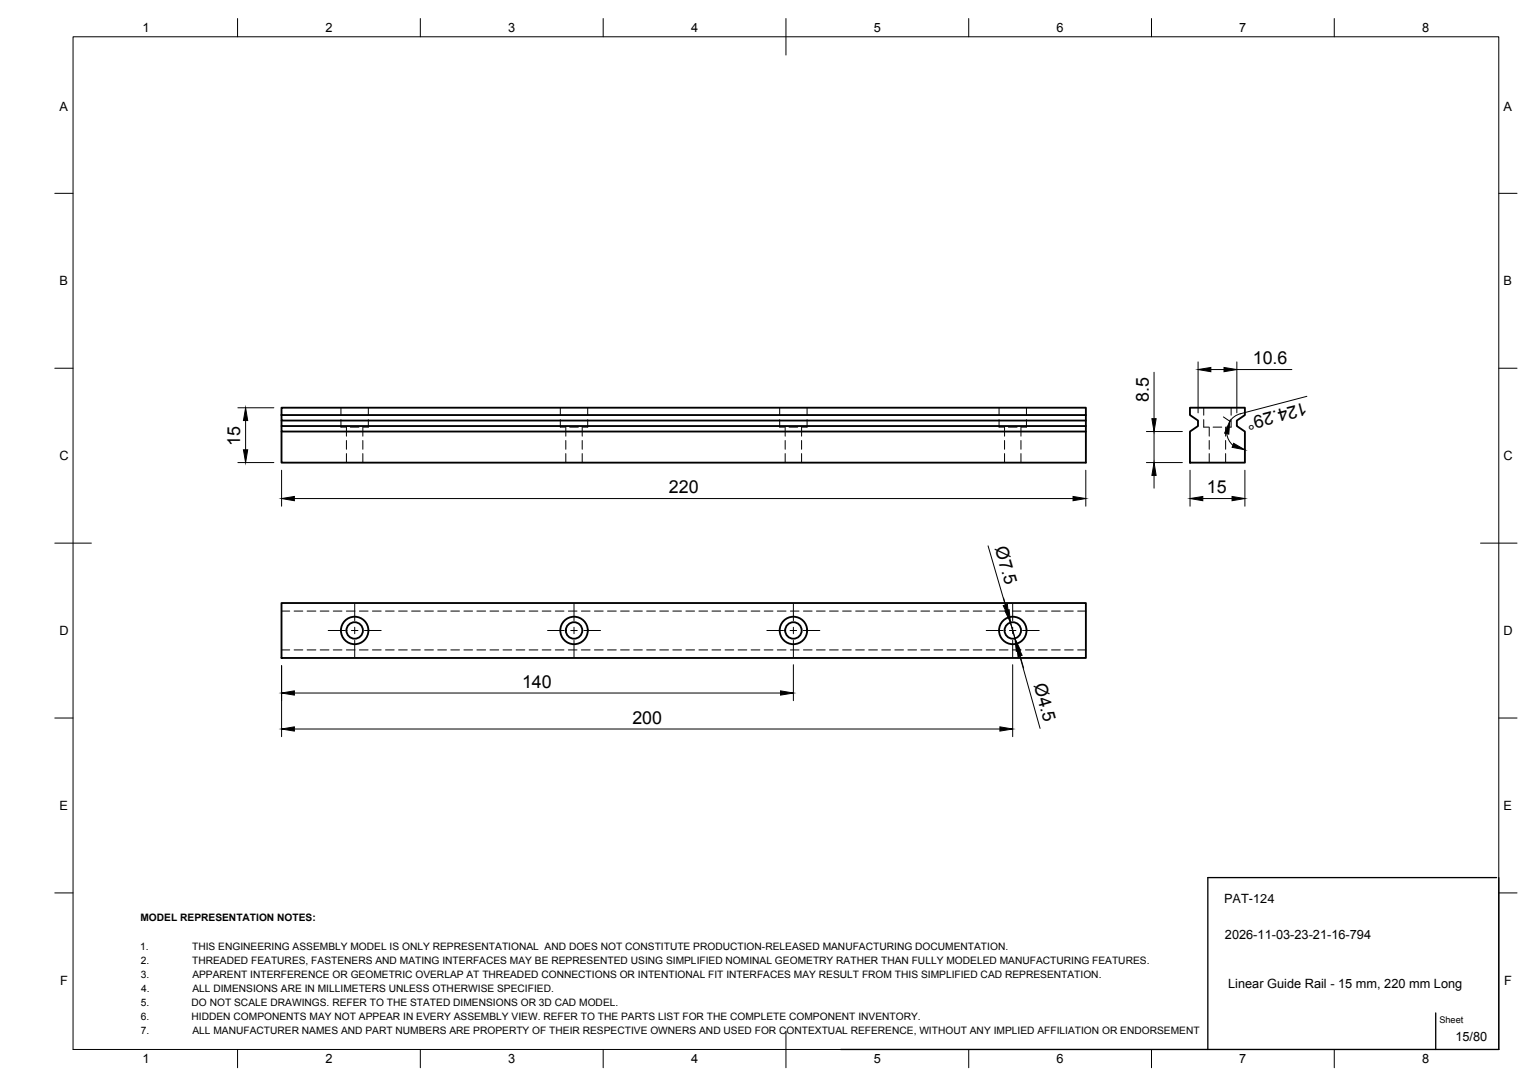
ISO-10303-21;
HEADER;
/* Generated by software containing ST-Developer
 * from STEP Tools, Inc. (www.steptools.com) 
 */

FILE_DESCRIPTION(
/* description */ ('XY cross-slide table'),
/* implementation_level */ '2;1');

FILE_NAME(
/* name */ 'Linear Guide Rail - 15 mm, 220 mm Long.step',
/* time_stamp */ '2026-10-28T03:22:46-07:00',
/* author */ (''),
/* organization */ (''),
/* preprocessor_version */ 'ST-DEVELOPER v20.2',
/* originating_system */ 'Autodesk Translation Framework v15.17.0.0',
/* authorisation */ '');

FILE_SCHEMA (('AUTOMOTIVE_DESIGN { 1 0 10303 214 3 1 1 }'));
ENDSEC;

DATA;
#10=MECHANICAL_DESIGN_GEOMETRIC_PRESENTATION_REPRESENTATION('',(#1680),#62984);
#1514=SHAPE_REPRESENTATION_RELATIONSHIP('SRR','None',#63362,#1597);
#1597=ADVANCED_BREP_SHAPE_REPRESENTATION('',(#1793),#62899);
#1680=STYLED_ITEM('',(#63905),#1793);
#1793=MANIFOLD_SOLID_BREP('Body1',#22974);
#1971=FACE_BOUND('',#4390,.T.);
#1972=FACE_BOUND('',#4393,.T.);
#1973=FACE_BOUND('',#4396,.T.);
#1974=FACE_BOUND('',#4399,.T.);
#1975=FACE_BOUND('',#4409,.T.);
#1976=FACE_BOUND('',#4410,.T.);
#1977=FACE_BOUND('',#4411,.T.);
#1978=FACE_BOUND('',#4412,.T.);
#1979=FACE_BOUND('',#4419,.T.);
#1980=FACE_BOUND('',#4420,.T.);
#1981=FACE_BOUND('',#4421,.T.);
#1982=FACE_BOUND('',#4422,.T.);
#2363=PLANE('',#24246);
#2364=PLANE('',#24251);
#2365=PLANE('',#24256);
#2366=PLANE('',#24261);
#2367=PLANE('',#24271);
#2368=PLANE('',#24272);
#2369=PLANE('',#24273);
#2370=PLANE('',#24274);
#2371=PLANE('',#24275);
#2372=PLANE('',#24276);
#2373=PLANE('',#24277);
#2374=PLANE('',#24278);
#2375=PLANE('',#24279);
#2376=PLANE('',#24280);
#2377=PLANE('',#24281);
#2378=PLANE('',#24282);
#2379=PLANE('',#24283);
#2380=PLANE('',#24284);
#2990=FACE_OUTER_BOUND('',#4388,.T.);
#2991=FACE_OUTER_BOUND('',#4389,.T.);
#2992=FACE_OUTER_BOUND('',#4391,.T.);
#2993=FACE_OUTER_BOUND('',#4392,.T.);
#2994=FACE_OUTER_BOUND('',#4394,.T.);
#2995=FACE_OUTER_BOUND('',#4395,.T.);
#2996=FACE_OUTER_BOUND('',#4397,.T.);
#2997=FACE_OUTER_BOUND('',#4398,.T.);
#2998=FACE_OUTER_BOUND('',#4400,.T.);
#2999=FACE_OUTER_BOUND('',#4401,.T.);
#3000=FACE_OUTER_BOUND('',#4402,.T.);
#3001=FACE_OUTER_BOUND('',#4403,.T.);
#3002=FACE_OUTER_BOUND('',#4404,.T.);
#3003=FACE_OUTER_BOUND('',#4405,.T.);
#3004=FACE_OUTER_BOUND('',#4406,.T.);
#3005=FACE_OUTER_BOUND('',#4407,.T.);
#3006=FACE_OUTER_BOUND('',#4408,.T.);
#3007=FACE_OUTER_BOUND('',#4413,.T.);
#3008=FACE_OUTER_BOUND('',#4414,.T.);
#3009=FACE_OUTER_BOUND('',#4415,.T.);
#3010=FACE_OUTER_BOUND('',#4416,.T.);
#3011=FACE_OUTER_BOUND('',#4417,.T.);
#3012=FACE_OUTER_BOUND('',#4418,.T.);
#3013=FACE_OUTER_BOUND('',#4423,.T.);
#3014=FACE_OUTER_BOUND('',#4424,.T.);
#3015=FACE_OUTER_BOUND('',#4425,.T.);
#4388=EDGE_LOOP('',(#15434,#15435,#15436,#15437));
#4389=EDGE_LOOP('',(#15438));
#4390=EDGE_LOOP('',(#15439));
#4391=EDGE_LOOP('',(#15440,#15441,#15442,#15443));
#4392=EDGE_LOOP('',(#15444));
#4393=EDGE_LOOP('',(#15445));
#4394=EDGE_LOOP('',(#15446,#15447,#15448,#15449));
#4395=EDGE_LOOP('',(#15450));
#4396=EDGE_LOOP('',(#15451));
#4397=EDGE_LOOP('',(#15452,#15453,#15454,#15455));
#4398=EDGE_LOOP('',(#15456));
#4399=EDGE_LOOP('',(#15457));
#4400=EDGE_LOOP('',(#15458,#15459,#15460,#15461));
#4401=EDGE_LOOP('',(#15462,#15463,#15464,#15465));
#4402=EDGE_LOOP('',(#15466,#15467,#15468,#15469));
#4403=EDGE_LOOP('',(#15470,#15471,#15472,#15473));
#4404=EDGE_LOOP('',(#15474,#15475,#15476,#15477));
#4405=EDGE_LOOP('',(#15478,#15479,#15480,#15481));
#4406=EDGE_LOOP('',(#15482,#15483,#15484,#15485));
#4407=EDGE_LOOP('',(#15486,#15487,#15488,#15489));
#4408=EDGE_LOOP('',(#15490,#15491,#15492,#15493));
#4409=EDGE_LOOP('',(#15494));
#4410=EDGE_LOOP('',(#15495));
#4411=EDGE_LOOP('',(#15496));
#4412=EDGE_LOOP('',(#15497));
#4413=EDGE_LOOP('',(#15498,#15499,#15500,#15501));
#4414=EDGE_LOOP('',(#15502,#15503,#15504,#15505));
#4415=EDGE_LOOP('',(#15506,#15507,#15508,#15509));
#4416=EDGE_LOOP('',(#15510,#15511,#15512,#15513));
#4417=EDGE_LOOP('',(#15514,#15515,#15516,#15517));
#4418=EDGE_LOOP('',(#15518,#15519,#15520,#15521));
#4419=EDGE_LOOP('',(#15522));
#4420=EDGE_LOOP('',(#15523));
#4421=EDGE_LOOP('',(#15524));
#4422=EDGE_LOOP('',(#15525));
#4423=EDGE_LOOP('',(#15526,#15527,#15528,#15529));
#4424=EDGE_LOOP('',(#15530,#15531,#15532,#15533,#15534,#15535,#15536,#15537,
#15538,#15539,#15540,#15541));
#4425=EDGE_LOOP('',(#15542,#15543,#15544,#15545,#15546,#15547,#15548,#15549,
#15550,#15551,#15552,#15553));
#6063=LINE('',#33448,#7550);
#6064=LINE('',#33457,#7551);
#6065=LINE('',#33466,#7552);
#6066=LINE('',#33475,#7553);
#6067=LINE('',#33483,#7554);
#6068=LINE('',#33487,#7555);
#6069=LINE('',#33491,#7556);
#6070=LINE('',#33495,#7557);
#6071=LINE('',#33499,#7558);
#6072=LINE('',#33501,#7559);
#6073=LINE('',#33503,#7560);
#6074=LINE('',#33504,#7561);
#6075=LINE('',#33507,#7562);
#6076=LINE('',#33509,#7563);
#6077=LINE('',#33510,#7564);
#6078=LINE('',#33513,#7565);
#6079=LINE('',#33515,#7566);
#6080=LINE('',#33516,#7567);
#6081=LINE('',#33519,#7568);
#6082=LINE('',#33521,#7569);
#6083=LINE('',#33522,#7570);
#6084=LINE('',#33525,#7571);
#6085=LINE('',#33527,#7572);
#6086=LINE('',#33528,#7573);
#6087=LINE('',#33531,#7574);
#6088=LINE('',#33533,#7575);
#6089=LINE('',#33534,#7576);
#6090=LINE('',#33537,#7577);
#6091=LINE('',#33539,#7578);
#6092=LINE('',#33540,#7579);
#6093=LINE('',#33543,#7580);
#6094=LINE('',#33545,#7581);
#6095=LINE('',#33546,#7582);
#6096=LINE('',#33549,#7583);
#6097=LINE('',#33551,#7584);
#6098=LINE('',#33552,#7585);
#6099=LINE('',#33555,#7586);
#6100=LINE('',#33557,#7587);
#6101=LINE('',#33558,#7588);
#6102=LINE('',#33561,#7589);
#6103=LINE('',#33563,#7590);
#6104=LINE('',#33564,#7591);
#6105=LINE('',#33566,#7592);
#6106=LINE('',#33567,#7593);
#7550=VECTOR('',#27108,0.375);
#7551=VECTOR('',#27119,0.375);
#7552=VECTOR('',#27130,0.375);
#7553=VECTOR('',#27141,0.375);
#7554=VECTOR('',#27152,0.225);
#7555=VECTOR('',#27157,0.225);
#7556=VECTOR('',#27162,0.225);
#7557=VECTOR('',#27167,0.225000000000001);
#7558=VECTOR('',#27170,1.);
#7559=VECTOR('',#27171,1.);
#7560=VECTOR('',#27172,1.);
#7561=VECTOR('',#27173,1.);
#7562=VECTOR('',#27176,1.);
#7563=VECTOR('',#27177,1.);
#7564=VECTOR('',#27178,1.);
#7565=VECTOR('',#27181,1.);
#7566=VECTOR('',#27182,1.);
#7567=VECTOR('',#27183,1.);
#7568=VECTOR('',#27186,1.);
#7569=VECTOR('',#27187,1.);
#7570=VECTOR('',#27188,1.);
#7571=VECTOR('',#27191,1.);
#7572=VECTOR('',#27192,1.);
#7573=VECTOR('',#27193,1.);
#7574=VECTOR('',#27196,1.);
#7575=VECTOR('',#27197,1.);
#7576=VECTOR('',#27198,1.);
#7577=VECTOR('',#27201,1.);
#7578=VECTOR('',#27202,1.);
#7579=VECTOR('',#27203,1.);
#7580=VECTOR('',#27206,1.);
#7581=VECTOR('',#27207,1.);
#7582=VECTOR('',#27208,1.);
#7583=VECTOR('',#27211,1.);
#7584=VECTOR('',#27212,1.);
#7585=VECTOR('',#27213,1.);
#7586=VECTOR('',#27216,1.);
#7587=VECTOR('',#27217,1.);
#7588=VECTOR('',#27218,1.);
#7589=VECTOR('',#27221,1.);
#7590=VECTOR('',#27222,1.);
#7591=VECTOR('',#27223,1.);
#7592=VECTOR('',#27226,1.);
#7593=VECTOR('',#27227,1.);
#8988=CIRCLE('',#24244,0.375);
#8989=CIRCLE('',#24245,0.375);
#8990=CIRCLE('',#24247,0.225);
#8991=CIRCLE('',#24249,0.375);
#8992=CIRCLE('',#24250,0.375);
#8993=CIRCLE('',#24252,0.225);
#8994=CIRCLE('',#24254,0.375);
#8995=CIRCLE('',#24255,0.375);
#8996=CIRCLE('',#24257,0.225);
#8997=CIRCLE('',#24259,0.375);
#8998=CIRCLE('',#24260,0.375);
#8999=CIRCLE('',#24262,0.225000000000001);
#9000=CIRCLE('',#24264,0.225);
#9001=CIRCLE('',#24266,0.225);
#9002=CIRCLE('',#24268,0.225);
#9003=CIRCLE('',#24270,0.225000000000001);
#9947=VERTEX_POINT('',#33445);
#9948=VERTEX_POINT('',#33447);
#9949=VERTEX_POINT('',#33451);
#9950=VERTEX_POINT('',#33454);
#9951=VERTEX_POINT('',#33456);
#9952=VERTEX_POINT('',#33460);
#9953=VERTEX_POINT('',#33463);
#9954=VERTEX_POINT('',#33465);
#9955=VERTEX_POINT('',#33469);
#9956=VERTEX_POINT('',#33472);
#9957=VERTEX_POINT('',#33474);
#9958=VERTEX_POINT('',#33478);
#9959=VERTEX_POINT('',#33481);
#9960=VERTEX_POINT('',#33485);
#9961=VERTEX_POINT('',#33489);
#9962=VERTEX_POINT('',#33493);
#9963=VERTEX_POINT('',#33497);
#9964=VERTEX_POINT('',#33498);
#9965=VERTEX_POINT('',#33500);
#9966=VERTEX_POINT('',#33502);
#9967=VERTEX_POINT('',#33506);
#9968=VERTEX_POINT('',#33508);
#9969=VERTEX_POINT('',#33512);
#9970=VERTEX_POINT('',#33514);
#9971=VERTEX_POINT('',#33518);
#9972=VERTEX_POINT('',#33520);
#9973=VERTEX_POINT('',#33524);
#9974=VERTEX_POINT('',#33526);
#9975=VERTEX_POINT('',#33530);
#9976=VERTEX_POINT('',#33532);
#9977=VERTEX_POINT('',#33536);
#9978=VERTEX_POINT('',#33538);
#9979=VERTEX_POINT('',#33542);
#9980=VERTEX_POINT('',#33544);
#9981=VERTEX_POINT('',#33548);
#9982=VERTEX_POINT('',#33550);
#9983=VERTEX_POINT('',#33554);
#9984=VERTEX_POINT('',#33556);
#9985=VERTEX_POINT('',#33560);
#9986=VERTEX_POINT('',#33562);
#12101=EDGE_CURVE('',#9947,#9947,#8988,.T.);
#12102=EDGE_CURVE('',#9947,#9948,#6063,.T.);
#12103=EDGE_CURVE('',#9948,#9948,#8989,.T.);
#12104=EDGE_CURVE('',#9949,#9949,#8990,.T.);
#12105=EDGE_CURVE('',#9950,#9950,#8991,.T.);
#12106=EDGE_CURVE('',#9950,#9951,#6064,.T.);
#12107=EDGE_CURVE('',#9951,#9951,#8992,.T.);
#12108=EDGE_CURVE('',#9952,#9952,#8993,.T.);
#12109=EDGE_CURVE('',#9953,#9953,#8994,.T.);
#12110=EDGE_CURVE('',#9953,#9954,#6065,.T.);
#12111=EDGE_CURVE('',#9954,#9954,#8995,.T.);
#12112=EDGE_CURVE('',#9955,#9955,#8996,.T.);
#12113=EDGE_CURVE('',#9956,#9956,#8997,.T.);
#12114=EDGE_CURVE('',#9956,#9957,#6066,.T.);
#12115=EDGE_CURVE('',#9957,#9957,#8998,.T.);
#12116=EDGE_CURVE('',#9958,#9958,#8999,.T.);
#12117=EDGE_CURVE('',#9959,#9959,#9000,.T.);
#12118=EDGE_CURVE('',#9959,#9949,#6067,.T.);
#12119=EDGE_CURVE('',#9960,#9960,#9001,.T.);
#12120=EDGE_CURVE('',#9960,#9952,#6068,.T.);
#12121=EDGE_CURVE('',#9961,#9961,#9002,.T.);
#12122=EDGE_CURVE('',#9961,#9955,#6069,.T.);
#12123=EDGE_CURVE('',#9962,#9962,#9003,.T.);
#12124=EDGE_CURVE('',#9962,#9958,#6070,.T.);
#12125=EDGE_CURVE('',#9963,#9964,#6071,.T.);
#12126=EDGE_CURVE('',#9964,#9965,#6072,.T.);
#12127=EDGE_CURVE('',#9966,#9965,#6073,.T.);
#12128=EDGE_CURVE('',#9963,#9966,#6074,.T.);
#12129=EDGE_CURVE('',#9967,#9963,#6075,.T.);
#12130=EDGE_CURVE('',#9968,#9966,#6076,.T.);
#12131=EDGE_CURVE('',#9967,#9968,#6077,.T.);
#12132=EDGE_CURVE('',#9969,#9967,#6078,.T.);
#12133=EDGE_CURVE('',#9970,#9968,#6079,.T.);
#12134=EDGE_CURVE('',#9969,#9970,#6080,.T.);
#12135=EDGE_CURVE('',#9971,#9969,#6081,.T.);
#12136=EDGE_CURVE('',#9972,#9970,#6082,.T.);
#12137=EDGE_CURVE('',#9971,#9972,#6083,.T.);
#12138=EDGE_CURVE('',#9973,#9971,#6084,.T.);
#12139=EDGE_CURVE('',#9974,#9972,#6085,.T.);
#12140=EDGE_CURVE('',#9973,#9974,#6086,.T.);
#12141=EDGE_CURVE('',#9975,#9973,#6087,.T.);
#12142=EDGE_CURVE('',#9976,#9974,#6088,.T.);
#12143=EDGE_CURVE('',#9975,#9976,#6089,.T.);
#12144=EDGE_CURVE('',#9977,#9975,#6090,.T.);
#12145=EDGE_CURVE('',#9978,#9976,#6091,.T.);
#12146=EDGE_CURVE('',#9977,#9978,#6092,.T.);
#12147=EDGE_CURVE('',#9979,#9977,#6093,.T.);
#12148=EDGE_CURVE('',#9980,#9978,#6094,.T.);
#12149=EDGE_CURVE('',#9979,#9980,#6095,.T.);
#12150=EDGE_CURVE('',#9981,#9979,#6096,.T.);
#12151=EDGE_CURVE('',#9982,#9980,#6097,.T.);
#12152=EDGE_CURVE('',#9981,#9982,#6098,.T.);
#12153=EDGE_CURVE('',#9983,#9981,#6099,.T.);
#12154=EDGE_CURVE('',#9984,#9982,#6100,.T.);
#12155=EDGE_CURVE('',#9983,#9984,#6101,.T.);
#12156=EDGE_CURVE('',#9985,#9983,#6102,.T.);
#12157=EDGE_CURVE('',#9986,#9984,#6103,.T.);
#12158=EDGE_CURVE('',#9985,#9986,#6104,.T.);
#12159=EDGE_CURVE('',#9964,#9985,#6105,.T.);
#12160=EDGE_CURVE('',#9965,#9986,#6106,.T.);
#15434=ORIENTED_EDGE('',*,*,#12101,.F.);
#15435=ORIENTED_EDGE('',*,*,#12102,.T.);
#15436=ORIENTED_EDGE('',*,*,#12103,.F.);
#15437=ORIENTED_EDGE('',*,*,#12102,.F.);
#15438=ORIENTED_EDGE('',*,*,#12101,.T.);
#15439=ORIENTED_EDGE('',*,*,#12104,.F.);
#15440=ORIENTED_EDGE('',*,*,#12105,.F.);
#15441=ORIENTED_EDGE('',*,*,#12106,.T.);
#15442=ORIENTED_EDGE('',*,*,#12107,.F.);
#15443=ORIENTED_EDGE('',*,*,#12106,.F.);
#15444=ORIENTED_EDGE('',*,*,#12105,.T.);
#15445=ORIENTED_EDGE('',*,*,#12108,.F.);
#15446=ORIENTED_EDGE('',*,*,#12109,.F.);
#15447=ORIENTED_EDGE('',*,*,#12110,.T.);
#15448=ORIENTED_EDGE('',*,*,#12111,.F.);
#15449=ORIENTED_EDGE('',*,*,#12110,.F.);
#15450=ORIENTED_EDGE('',*,*,#12109,.T.);
#15451=ORIENTED_EDGE('',*,*,#12112,.F.);
#15452=ORIENTED_EDGE('',*,*,#12113,.F.);
#15453=ORIENTED_EDGE('',*,*,#12114,.T.);
#15454=ORIENTED_EDGE('',*,*,#12115,.F.);
#15455=ORIENTED_EDGE('',*,*,#12114,.F.);
#15456=ORIENTED_EDGE('',*,*,#12113,.T.);
#15457=ORIENTED_EDGE('',*,*,#12116,.F.);
#15458=ORIENTED_EDGE('',*,*,#12117,.F.);
#15459=ORIENTED_EDGE('',*,*,#12118,.T.);
#15460=ORIENTED_EDGE('',*,*,#12104,.T.);
#15461=ORIENTED_EDGE('',*,*,#12118,.F.);
#15462=ORIENTED_EDGE('',*,*,#12119,.F.);
#15463=ORIENTED_EDGE('',*,*,#12120,.T.);
#15464=ORIENTED_EDGE('',*,*,#12108,.T.);
#15465=ORIENTED_EDGE('',*,*,#12120,.F.);
#15466=ORIENTED_EDGE('',*,*,#12121,.F.);
#15467=ORIENTED_EDGE('',*,*,#12122,.T.);
#15468=ORIENTED_EDGE('',*,*,#12112,.T.);
#15469=ORIENTED_EDGE('',*,*,#12122,.F.);
#15470=ORIENTED_EDGE('',*,*,#12123,.F.);
#15471=ORIENTED_EDGE('',*,*,#12124,.T.);
#15472=ORIENTED_EDGE('',*,*,#12116,.T.);
#15473=ORIENTED_EDGE('',*,*,#12124,.F.);
#15474=ORIENTED_EDGE('',*,*,#12125,.T.);
#15475=ORIENTED_EDGE('',*,*,#12126,.T.);
#15476=ORIENTED_EDGE('',*,*,#12127,.F.);
#15477=ORIENTED_EDGE('',*,*,#12128,.F.);
#15478=ORIENTED_EDGE('',*,*,#12129,.T.);
#15479=ORIENTED_EDGE('',*,*,#12128,.T.);
#15480=ORIENTED_EDGE('',*,*,#12130,.F.);
#15481=ORIENTED_EDGE('',*,*,#12131,.F.);
#15482=ORIENTED_EDGE('',*,*,#12132,.T.);
#15483=ORIENTED_EDGE('',*,*,#12131,.T.);
#15484=ORIENTED_EDGE('',*,*,#12133,.F.);
#15485=ORIENTED_EDGE('',*,*,#12134,.F.);
#15486=ORIENTED_EDGE('',*,*,#12135,.T.);
#15487=ORIENTED_EDGE('',*,*,#12134,.T.);
#15488=ORIENTED_EDGE('',*,*,#12136,.F.);
#15489=ORIENTED_EDGE('',*,*,#12137,.F.);
#15490=ORIENTED_EDGE('',*,*,#12138,.T.);
#15491=ORIENTED_EDGE('',*,*,#12137,.T.);
#15492=ORIENTED_EDGE('',*,*,#12139,.F.);
#15493=ORIENTED_EDGE('',*,*,#12140,.F.);
#15494=ORIENTED_EDGE('',*,*,#12115,.T.);
#15495=ORIENTED_EDGE('',*,*,#12111,.T.);
#15496=ORIENTED_EDGE('',*,*,#12107,.T.);
#15497=ORIENTED_EDGE('',*,*,#12103,.T.);
#15498=ORIENTED_EDGE('',*,*,#12141,.T.);
#15499=ORIENTED_EDGE('',*,*,#12140,.T.);
#15500=ORIENTED_EDGE('',*,*,#12142,.F.);
#15501=ORIENTED_EDGE('',*,*,#12143,.F.);
#15502=ORIENTED_EDGE('',*,*,#12144,.T.);
#15503=ORIENTED_EDGE('',*,*,#12143,.T.);
#15504=ORIENTED_EDGE('',*,*,#12145,.F.);
#15505=ORIENTED_EDGE('',*,*,#12146,.F.);
#15506=ORIENTED_EDGE('',*,*,#12147,.T.);
#15507=ORIENTED_EDGE('',*,*,#12146,.T.);
#15508=ORIENTED_EDGE('',*,*,#12148,.F.);
#15509=ORIENTED_EDGE('',*,*,#12149,.F.);
#15510=ORIENTED_EDGE('',*,*,#12150,.T.);
#15511=ORIENTED_EDGE('',*,*,#12149,.T.);
#15512=ORIENTED_EDGE('',*,*,#12151,.F.);
#15513=ORIENTED_EDGE('',*,*,#12152,.F.);
#15514=ORIENTED_EDGE('',*,*,#12153,.T.);
#15515=ORIENTED_EDGE('',*,*,#12152,.T.);
#15516=ORIENTED_EDGE('',*,*,#12154,.F.);
#15517=ORIENTED_EDGE('',*,*,#12155,.F.);
#15518=ORIENTED_EDGE('',*,*,#12156,.T.);
#15519=ORIENTED_EDGE('',*,*,#12155,.T.);
#15520=ORIENTED_EDGE('',*,*,#12157,.F.);
#15521=ORIENTED_EDGE('',*,*,#12158,.F.);
#15522=ORIENTED_EDGE('',*,*,#12117,.T.);
#15523=ORIENTED_EDGE('',*,*,#12119,.T.);
#15524=ORIENTED_EDGE('',*,*,#12121,.T.);
#15525=ORIENTED_EDGE('',*,*,#12123,.T.);
#15526=ORIENTED_EDGE('',*,*,#12159,.T.);
#15527=ORIENTED_EDGE('',*,*,#12158,.T.);
#15528=ORIENTED_EDGE('',*,*,#12160,.F.);
#15529=ORIENTED_EDGE('',*,*,#12126,.F.);
#15530=ORIENTED_EDGE('',*,*,#12160,.T.);
#15531=ORIENTED_EDGE('',*,*,#12157,.T.);
#15532=ORIENTED_EDGE('',*,*,#12154,.T.);
#15533=ORIENTED_EDGE('',*,*,#12151,.T.);
#15534=ORIENTED_EDGE('',*,*,#12148,.T.);
#15535=ORIENTED_EDGE('',*,*,#12145,.T.);
#15536=ORIENTED_EDGE('',*,*,#12142,.T.);
#15537=ORIENTED_EDGE('',*,*,#12139,.T.);
#15538=ORIENTED_EDGE('',*,*,#12136,.T.);
#15539=ORIENTED_EDGE('',*,*,#12133,.T.);
#15540=ORIENTED_EDGE('',*,*,#12130,.T.);
#15541=ORIENTED_EDGE('',*,*,#12127,.T.);
#15542=ORIENTED_EDGE('',*,*,#12159,.F.);
#15543=ORIENTED_EDGE('',*,*,#12125,.F.);
#15544=ORIENTED_EDGE('',*,*,#12129,.F.);
#15545=ORIENTED_EDGE('',*,*,#12132,.F.);
#15546=ORIENTED_EDGE('',*,*,#12135,.F.);
#15547=ORIENTED_EDGE('',*,*,#12138,.F.);
#15548=ORIENTED_EDGE('',*,*,#12141,.F.);
#15549=ORIENTED_EDGE('',*,*,#12144,.F.);
#15550=ORIENTED_EDGE('',*,*,#12147,.F.);
#15551=ORIENTED_EDGE('',*,*,#12150,.F.);
#15552=ORIENTED_EDGE('',*,*,#12153,.F.);
#15553=ORIENTED_EDGE('',*,*,#12156,.F.);
#21094=CYLINDRICAL_SURFACE('',#24243,0.375);
#21095=CYLINDRICAL_SURFACE('',#24248,0.375);
#21096=CYLINDRICAL_SURFACE('',#24253,0.375);
#21097=CYLINDRICAL_SURFACE('',#24258,0.375);
#21098=CYLINDRICAL_SURFACE('',#24263,0.225);
#21099=CYLINDRICAL_SURFACE('',#24265,0.225);
#21100=CYLINDRICAL_SURFACE('',#24267,0.225);
#21101=CYLINDRICAL_SURFACE('',#24269,0.225000000000001);
#21771=ADVANCED_FACE('',(#2990),#21094,.F.);
#21772=ADVANCED_FACE('',(#2991,#1971),#2363,.T.);
#21773=ADVANCED_FACE('',(#2992),#21095,.F.);
#21774=ADVANCED_FACE('',(#2993,#1972),#2364,.T.);
#21775=ADVANCED_FACE('',(#2994),#21096,.F.);
#21776=ADVANCED_FACE('',(#2995,#1973),#2365,.T.);
#21777=ADVANCED_FACE('',(#2996),#21097,.F.);
#21778=ADVANCED_FACE('',(#2997,#1974),#2366,.T.);
#21779=ADVANCED_FACE('',(#2998),#21098,.F.);
#21780=ADVANCED_FACE('',(#2999),#21099,.F.);
#21781=ADVANCED_FACE('',(#3000),#21100,.F.);
#21782=ADVANCED_FACE('',(#3001),#21101,.F.);
#21783=ADVANCED_FACE('',(#3002),#2367,.T.);
#21784=ADVANCED_FACE('',(#3003),#2368,.T.);
#21785=ADVANCED_FACE('',(#3004),#2369,.T.);
#21786=ADVANCED_FACE('',(#3005),#2370,.T.);
#21787=ADVANCED_FACE('',(#3006,#1975,#1976,#1977,#1978),#2371,.T.);
#21788=ADVANCED_FACE('',(#3007),#2372,.T.);
#21789=ADVANCED_FACE('',(#3008),#2373,.T.);
#21790=ADVANCED_FACE('',(#3009),#2374,.T.);
#21791=ADVANCED_FACE('',(#3010),#2375,.T.);
#21792=ADVANCED_FACE('',(#3011),#2376,.T.);
#21793=ADVANCED_FACE('',(#3012,#1979,#1980,#1981,#1982),#2377,.T.);
#21794=ADVANCED_FACE('',(#3013),#2378,.T.);
#21795=ADVANCED_FACE('',(#3014),#2379,.T.);
#21796=ADVANCED_FACE('',(#3015),#2380,.F.);
#22974=CLOSED_SHELL('',(#21771,#21772,#21773,#21774,#21775,#21776,#21777,
#21778,#21779,#21780,#21781,#21782,#21783,#21784,#21785,#21786,#21787,#21788,
#21789,#21790,#21791,#21792,#21793,#21794,#21795,#21796));
#24242=AXIS2_PLACEMENT_3D('',#33443,#27102,#27103);
#24243=AXIS2_PLACEMENT_3D('',#33444,#27104,#27105);
#24244=AXIS2_PLACEMENT_3D('',#33446,#27106,#27107);
#24245=AXIS2_PLACEMENT_3D('',#33449,#27109,#27110);
#24246=AXIS2_PLACEMENT_3D('',#33450,#27111,#27112);
#24247=AXIS2_PLACEMENT_3D('',#33452,#27113,#27114);
#24248=AXIS2_PLACEMENT_3D('',#33453,#27115,#27116);
#24249=AXIS2_PLACEMENT_3D('',#33455,#27117,#27118);
#24250=AXIS2_PLACEMENT_3D('',#33458,#27120,#27121);
#24251=AXIS2_PLACEMENT_3D('',#33459,#27122,#27123);
#24252=AXIS2_PLACEMENT_3D('',#33461,#27124,#27125);
#24253=AXIS2_PLACEMENT_3D('',#33462,#27126,#27127);
#24254=AXIS2_PLACEMENT_3D('',#33464,#27128,#27129);
#24255=AXIS2_PLACEMENT_3D('',#33467,#27131,#27132);
#24256=AXIS2_PLACEMENT_3D('',#33468,#27133,#27134);
#24257=AXIS2_PLACEMENT_3D('',#33470,#27135,#27136);
#24258=AXIS2_PLACEMENT_3D('',#33471,#27137,#27138);
#24259=AXIS2_PLACEMENT_3D('',#33473,#27139,#27140);
#24260=AXIS2_PLACEMENT_3D('',#33476,#27142,#27143);
#24261=AXIS2_PLACEMENT_3D('',#33477,#27144,#27145);
#24262=AXIS2_PLACEMENT_3D('',#33479,#27146,#27147);
#24263=AXIS2_PLACEMENT_3D('',#33480,#27148,#27149);
#24264=AXIS2_PLACEMENT_3D('',#33482,#27150,#27151);
#24265=AXIS2_PLACEMENT_3D('',#33484,#27153,#27154);
#24266=AXIS2_PLACEMENT_3D('',#33486,#27155,#27156);
#24267=AXIS2_PLACEMENT_3D('',#33488,#27158,#27159);
#24268=AXIS2_PLACEMENT_3D('',#33490,#27160,#27161);
#24269=AXIS2_PLACEMENT_3D('',#33492,#27163,#27164);
#24270=AXIS2_PLACEMENT_3D('',#33494,#27165,#27166);
#24271=AXIS2_PLACEMENT_3D('',#33496,#27168,#27169);
#24272=AXIS2_PLACEMENT_3D('',#33505,#27174,#27175);
#24273=AXIS2_PLACEMENT_3D('',#33511,#27179,#27180);
#24274=AXIS2_PLACEMENT_3D('',#33517,#27184,#27185);
#24275=AXIS2_PLACEMENT_3D('',#33523,#27189,#27190);
#24276=AXIS2_PLACEMENT_3D('',#33529,#27194,#27195);
#24277=AXIS2_PLACEMENT_3D('',#33535,#27199,#27200);
#24278=AXIS2_PLACEMENT_3D('',#33541,#27204,#27205);
#24279=AXIS2_PLACEMENT_3D('',#33547,#27209,#27210);
#24280=AXIS2_PLACEMENT_3D('',#33553,#27214,#27215);
#24281=AXIS2_PLACEMENT_3D('',#33559,#27219,#27220);
#24282=AXIS2_PLACEMENT_3D('',#33565,#27224,#27225);
#24283=AXIS2_PLACEMENT_3D('',#33568,#27228,#27229);
#24284=AXIS2_PLACEMENT_3D('',#33569,#27230,#27231);
#27102=DIRECTION('axis',(0.,0.,1.));
#27103=DIRECTION('refdir',(1.,0.,0.));
#27104=DIRECTION('center_axis',(0.,0.,1.));
#27105=DIRECTION('ref_axis',(1.,0.,0.));
#27106=DIRECTION('center_axis',(0.,0.,1.));
#27107=DIRECTION('ref_axis',(1.,0.,0.));
#27108=DIRECTION('',(0.,0.,1.));
#27109=DIRECTION('center_axis',(0.,0.,-1.));
#27110=DIRECTION('ref_axis',(1.,0.,0.));
#27111=DIRECTION('center_axis',(0.,0.,1.));
#27112=DIRECTION('ref_axis',(1.,0.,0.));
#27113=DIRECTION('center_axis',(0.,0.,1.));
#27114=DIRECTION('ref_axis',(1.,0.,0.));
#27115=DIRECTION('center_axis',(0.,0.,1.));
#27116=DIRECTION('ref_axis',(1.,0.,0.));
#27117=DIRECTION('center_axis',(0.,0.,1.));
#27118=DIRECTION('ref_axis',(1.,0.,0.));
#27119=DIRECTION('',(0.,0.,1.));
#27120=DIRECTION('center_axis',(0.,0.,-1.));
#27121=DIRECTION('ref_axis',(1.,0.,0.));
#27122=DIRECTION('center_axis',(0.,0.,1.));
#27123=DIRECTION('ref_axis',(1.,0.,0.));
#27124=DIRECTION('center_axis',(0.,0.,1.));
#27125=DIRECTION('ref_axis',(1.,0.,0.));
#27126=DIRECTION('center_axis',(0.,0.,1.));
#27127=DIRECTION('ref_axis',(1.,0.,0.));
#27128=DIRECTION('center_axis',(0.,0.,1.));
#27129=DIRECTION('ref_axis',(1.,0.,0.));
#27130=DIRECTION('',(0.,0.,1.));
#27131=DIRECTION('center_axis',(0.,0.,-1.));
#27132=DIRECTION('ref_axis',(1.,0.,0.));
#27133=DIRECTION('center_axis',(0.,0.,1.));
#27134=DIRECTION('ref_axis',(1.,0.,0.));
#27135=DIRECTION('center_axis',(0.,0.,1.));
#27136=DIRECTION('ref_axis',(1.,0.,0.));
#27137=DIRECTION('center_axis',(0.,0.,1.));
#27138=DIRECTION('ref_axis',(1.,0.,0.));
#27139=DIRECTION('center_axis',(0.,0.,1.));
#27140=DIRECTION('ref_axis',(1.,0.,0.));
#27141=DIRECTION('',(0.,0.,1.));
#27142=DIRECTION('center_axis',(0.,0.,-1.));
#27143=DIRECTION('ref_axis',(1.,0.,0.));
#27144=DIRECTION('center_axis',(0.,0.,1.));
#27145=DIRECTION('ref_axis',(1.,0.,0.));
#27146=DIRECTION('center_axis',(0.,0.,1.));
#27147=DIRECTION('ref_axis',(1.,0.,0.));
#27148=DIRECTION('center_axis',(0.,0.,1.));
#27149=DIRECTION('ref_axis',(1.,0.,0.));
#27150=DIRECTION('center_axis',(0.,0.,1.));
#27151=DIRECTION('ref_axis',(1.,0.,0.));
#27152=DIRECTION('',(0.,0.,1.));
#27153=DIRECTION('center_axis',(0.,0.,1.));
#27154=DIRECTION('ref_axis',(1.,0.,0.));
#27155=DIRECTION('center_axis',(0.,0.,1.));
#27156=DIRECTION('ref_axis',(1.,0.,0.));
#27157=DIRECTION('',(0.,0.,1.));
#27158=DIRECTION('center_axis',(0.,0.,1.));
#27159=DIRECTION('ref_axis',(1.,0.,0.));
#27160=DIRECTION('center_axis',(0.,0.,1.));
#27161=DIRECTION('ref_axis',(1.,0.,0.));
#27162=DIRECTION('',(0.,0.,1.));
#27163=DIRECTION('center_axis',(0.,0.,1.));
#27164=DIRECTION('ref_axis',(1.,0.,0.));
#27165=DIRECTION('center_axis',(0.,0.,1.));
#27166=DIRECTION('ref_axis',(1.,0.,0.));
#27167=DIRECTION('',(0.,0.,1.));
#27168=DIRECTION('center_axis',(0.,-0.56333682464151,0.826227342807548));
#27169=DIRECTION('ref_axis',(0.,-0.826227342807548,-0.56333682464151));
#27170=DIRECTION('',(0.,-0.826227342807548,-0.56333682464151));
#27171=DIRECTION('',(1.,0.,0.));
#27172=DIRECTION('',(0.,-0.826227342807548,-0.56333682464151));
#27173=DIRECTION('',(1.,0.,0.));
#27174=DIRECTION('center_axis',(0.,-1.,0.));
#27175=DIRECTION('ref_axis',(0.,0.,-1.));
#27176=DIRECTION('',(0.,0.,-1.));
#27177=DIRECTION('',(0.,0.,-1.));
#27178=DIRECTION('',(1.,0.,0.));
#27179=DIRECTION('center_axis',(0.,-0.56333682464151,-0.826227342807548));
#27180=DIRECTION('ref_axis',(0.,0.826227342807548,-0.56333682464151));
#27181=DIRECTION('',(0.,0.826227342807548,-0.56333682464151));
#27182=DIRECTION('',(0.,0.826227342807548,-0.56333682464151));
#27183=DIRECTION('',(1.,0.,0.));
#27184=DIRECTION('center_axis',(0.,-1.,0.));
#27185=DIRECTION('ref_axis',(0.,0.,-1.));
#27186=DIRECTION('',(0.,0.,-1.));
#27187=DIRECTION('',(0.,0.,-1.));
#27188=DIRECTION('',(1.,0.,0.));
#27189=DIRECTION('center_axis',(0.,0.,1.));
#27190=DIRECTION('ref_axis',(0.,-1.,0.));
#27191=DIRECTION('',(0.,-1.,0.));
#27192=DIRECTION('',(0.,-1.,0.));
#27193=DIRECTION('',(1.,0.,0.));
#27194=DIRECTION('center_axis',(0.,1.,0.));
#27195=DIRECTION('ref_axis',(0.,0.,1.));
#27196=DIRECTION('',(0.,0.,1.));
#27197=DIRECTION('',(0.,0.,1.));
#27198=DIRECTION('',(1.,0.,0.));
#27199=DIRECTION('center_axis',(0.,0.56333682464151,-0.826227342807548));
#27200=DIRECTION('ref_axis',(0.,0.826227342807548,0.56333682464151));
#27201=DIRECTION('',(0.,0.826227342807548,0.56333682464151));
#27202=DIRECTION('',(0.,0.826227342807548,0.56333682464151));
#27203=DIRECTION('',(1.,0.,0.));
#27204=DIRECTION('center_axis',(0.,1.,0.));
#27205=DIRECTION('ref_axis',(0.,0.,1.));
#27206=DIRECTION('',(0.,0.,1.));
#27207=DIRECTION('',(0.,0.,1.));
#27208=DIRECTION('',(1.,0.,0.));
#27209=DIRECTION('center_axis',(0.,0.56333682464151,0.826227342807548));
#27210=DIRECTION('ref_axis',(0.,-0.826227342807548,0.56333682464151));
#27211=DIRECTION('',(0.,-0.826227342807548,0.56333682464151));
#27212=DIRECTION('',(0.,-0.826227342807548,0.56333682464151));
#27213=DIRECTION('',(1.,0.,0.));
#27214=DIRECTION('center_axis',(0.,1.,0.));
#27215=DIRECTION('ref_axis',(0.,0.,1.));
#27216=DIRECTION('',(0.,0.,1.));
#27217=DIRECTION('',(0.,0.,1.));
#27218=DIRECTION('',(1.,0.,0.));
#27219=DIRECTION('center_axis',(0.,0.,-1.));
#27220=DIRECTION('ref_axis',(0.,1.,0.));
#27221=DIRECTION('',(0.,1.,0.));
#27222=DIRECTION('',(0.,1.,0.));
#27223=DIRECTION('',(1.,0.,0.));
#27224=DIRECTION('center_axis',(0.,-1.,0.));
#27225=DIRECTION('ref_axis',(0.,0.,-1.));
#27226=DIRECTION('',(0.,0.,-1.));
#27227=DIRECTION('',(0.,0.,-1.));
#27228=DIRECTION('center_axis',(1.,0.,0.));
#27229=DIRECTION('ref_axis',(0.,0.,-1.));
#27230=DIRECTION('center_axis',(1.,0.,0.));
#27231=DIRECTION('ref_axis',(0.,0.,-1.));
#33443=CARTESIAN_POINT('',(0.,0.,0.));
#33444=CARTESIAN_POINT('Origin',(14.,0.,0.97));
#33445=CARTESIAN_POINT('',(13.625,-4.59242549680257E-17,0.97));
#33446=CARTESIAN_POINT('Origin',(14.,0.,0.97));
#33447=CARTESIAN_POINT('',(13.625,4.59242549680257E-17,1.5));
#33448=CARTESIAN_POINT('',(13.625,-4.59242549680257E-17,0.97));
#33449=CARTESIAN_POINT('Origin',(14.,0.,1.5));
#33450=CARTESIAN_POINT('Origin',(14.,0.,0.97));
#33451=CARTESIAN_POINT('',(13.775,-2.75545529808154E-17,0.97));
#33452=CARTESIAN_POINT('Origin',(14.,0.,0.97));
#33453=CARTESIAN_POINT('Origin',(8.,0.,0.97));
#33454=CARTESIAN_POINT('',(7.625,-4.59242549680257E-17,0.97));
#33455=CARTESIAN_POINT('Origin',(8.,0.,0.97));
#33456=CARTESIAN_POINT('',(7.625,4.59242549680257E-17,1.5));
#33457=CARTESIAN_POINT('',(7.625,-4.59242549680257E-17,0.97));
#33458=CARTESIAN_POINT('Origin',(8.,0.,1.5));
#33459=CARTESIAN_POINT('Origin',(8.,0.,0.97));
#33460=CARTESIAN_POINT('',(7.775,-2.75545529808154E-17,0.97));
#33461=CARTESIAN_POINT('Origin',(8.,0.,0.97));
#33462=CARTESIAN_POINT('Origin',(2.,0.,0.97));
#33463=CARTESIAN_POINT('',(1.625,-4.59242549680257E-17,0.97));
#33464=CARTESIAN_POINT('Origin',(2.,0.,0.97));
#33465=CARTESIAN_POINT('',(1.625,4.59242549680257E-17,1.5));
#33466=CARTESIAN_POINT('',(1.625,-4.59242549680257E-17,0.97));
#33467=CARTESIAN_POINT('Origin',(2.,0.,1.5));
#33468=CARTESIAN_POINT('Origin',(2.,0.,0.97));
#33469=CARTESIAN_POINT('',(1.775,-2.75545529808155E-17,0.97));
#33470=CARTESIAN_POINT('Origin',(2.,0.,0.97));
#33471=CARTESIAN_POINT('Origin',(20.,0.,0.97));
#33472=CARTESIAN_POINT('',(19.625,-4.59242549680257E-17,0.97));
#33473=CARTESIAN_POINT('Origin',(20.,0.,0.97));
#33474=CARTESIAN_POINT('',(19.625,4.59242549680257E-17,1.5));
#33475=CARTESIAN_POINT('',(19.625,-4.59242549680257E-17,0.97));
#33476=CARTESIAN_POINT('Origin',(20.,0.,1.5));
#33477=CARTESIAN_POINT('Origin',(20.,0.,0.97));
#33478=CARTESIAN_POINT('',(19.775,-2.75545529808156E-17,0.97));
#33479=CARTESIAN_POINT('Origin',(20.,0.,0.97));
#33480=CARTESIAN_POINT('Origin',(14.,0.,-0.1));
#33481=CARTESIAN_POINT('',(13.775,-2.75545529808154E-17,0.));
#33482=CARTESIAN_POINT('Origin',(14.,0.,0.));
#33483=CARTESIAN_POINT('',(13.775,-2.75545529808154E-17,-0.1));
#33484=CARTESIAN_POINT('Origin',(8.,0.,-0.1));
#33485=CARTESIAN_POINT('',(7.775,-2.75545529808154E-17,0.));
#33486=CARTESIAN_POINT('Origin',(8.,0.,0.));
#33487=CARTESIAN_POINT('',(7.775,-2.75545529808154E-17,-0.1));
#33488=CARTESIAN_POINT('Origin',(2.,0.,-0.1));
#33489=CARTESIAN_POINT('',(1.775,-2.75545529808155E-17,0.));
#33490=CARTESIAN_POINT('Origin',(2.,0.,0.));
#33491=CARTESIAN_POINT('',(1.775,-2.75545529808155E-17,-0.1));
#33492=CARTESIAN_POINT('Origin',(20.,0.,-0.1));
#33493=CARTESIAN_POINT('',(19.775,-2.75545529808156E-17,0.));
#33494=CARTESIAN_POINT('Origin',(20.,0.,0.));
#33495=CARTESIAN_POINT('',(19.775,-2.75545529808156E-17,-0.1));
#33496=CARTESIAN_POINT('Origin',(0.,-0.53,1.));
#33497=CARTESIAN_POINT('',(0.,-0.53,1.));
#33498=CARTESIAN_POINT('',(0.,-0.75,0.85));
#33499=CARTESIAN_POINT('',(0.,-0.53,1.));
#33500=CARTESIAN_POINT('',(22.,-0.75,0.85));
#33501=CARTESIAN_POINT('',(0.,-0.75,0.85));
#33502=CARTESIAN_POINT('',(22.,-0.53,1.));
#33503=CARTESIAN_POINT('',(22.,-0.53,1.));
#33504=CARTESIAN_POINT('',(0.,-0.53,1.));
#33505=CARTESIAN_POINT('Origin',(0.,-0.53,1.15));
#33506=CARTESIAN_POINT('',(0.,-0.53,1.15));
#33507=CARTESIAN_POINT('',(0.,-0.53,1.15));
#33508=CARTESIAN_POINT('',(22.,-0.53,1.15));
#33509=CARTESIAN_POINT('',(22.,-0.53,1.15));
#33510=CARTESIAN_POINT('',(0.,-0.53,1.15));
#33511=CARTESIAN_POINT('Origin',(0.,-0.75,1.3));
#33512=CARTESIAN_POINT('',(0.,-0.75,1.3));
#33513=CARTESIAN_POINT('',(0.,-0.75,1.3));
#33514=CARTESIAN_POINT('',(22.,-0.75,1.3));
#33515=CARTESIAN_POINT('',(22.,-0.75,1.3));
#33516=CARTESIAN_POINT('',(0.,-0.75,1.3));
#33517=CARTESIAN_POINT('Origin',(0.,-0.75,1.5));
#33518=CARTESIAN_POINT('',(0.,-0.75,1.5));
#33519=CARTESIAN_POINT('',(0.,-0.75,1.5));
#33520=CARTESIAN_POINT('',(22.,-0.75,1.5));
#33521=CARTESIAN_POINT('',(22.,-0.75,1.5));
#33522=CARTESIAN_POINT('',(0.,-0.75,1.5));
#33523=CARTESIAN_POINT('Origin',(0.,0.75,1.5));
#33524=CARTESIAN_POINT('',(0.,0.75,1.5));
#33525=CARTESIAN_POINT('',(0.,0.75,1.5));
#33526=CARTESIAN_POINT('',(22.,0.75,1.5));
#33527=CARTESIAN_POINT('',(22.,0.75,1.5));
#33528=CARTESIAN_POINT('',(0.,0.75,1.5));
#33529=CARTESIAN_POINT('Origin',(0.,0.75,1.3));
#33530=CARTESIAN_POINT('',(0.,0.75,1.3));
#33531=CARTESIAN_POINT('',(0.,0.75,1.3));
#33532=CARTESIAN_POINT('',(22.,0.75,1.3));
#33533=CARTESIAN_POINT('',(22.,0.75,1.3));
#33534=CARTESIAN_POINT('',(0.,0.75,1.3));
#33535=CARTESIAN_POINT('Origin',(0.,0.53,1.15));
#33536=CARTESIAN_POINT('',(0.,0.53,1.15));
#33537=CARTESIAN_POINT('',(0.,0.53,1.15));
#33538=CARTESIAN_POINT('',(22.,0.53,1.15));
#33539=CARTESIAN_POINT('',(22.,0.53,1.15));
#33540=CARTESIAN_POINT('',(0.,0.53,1.15));
#33541=CARTESIAN_POINT('Origin',(0.,0.53,1.));
#33542=CARTESIAN_POINT('',(0.,0.53,1.));
#33543=CARTESIAN_POINT('',(0.,0.53,1.));
#33544=CARTESIAN_POINT('',(22.,0.53,1.));
#33545=CARTESIAN_POINT('',(22.,0.53,1.));
#33546=CARTESIAN_POINT('',(0.,0.53,1.));
#33547=CARTESIAN_POINT('Origin',(0.,0.75,0.85));
#33548=CARTESIAN_POINT('',(0.,0.75,0.85));
#33549=CARTESIAN_POINT('',(0.,0.75,0.85));
#33550=CARTESIAN_POINT('',(22.,0.75,0.85));
#33551=CARTESIAN_POINT('',(22.,0.75,0.85));
#33552=CARTESIAN_POINT('',(0.,0.75,0.85));
#33553=CARTESIAN_POINT('Origin',(0.,0.75,0.));
#33554=CARTESIAN_POINT('',(0.,0.75,0.));
#33555=CARTESIAN_POINT('',(0.,0.75,0.));
#33556=CARTESIAN_POINT('',(22.,0.75,0.));
#33557=CARTESIAN_POINT('',(22.,0.75,0.));
#33558=CARTESIAN_POINT('',(0.,0.75,0.));
#33559=CARTESIAN_POINT('Origin',(0.,-0.75,0.));
#33560=CARTESIAN_POINT('',(0.,-0.75,0.));
#33561=CARTESIAN_POINT('',(0.,-0.75,0.));
#33562=CARTESIAN_POINT('',(22.,-0.75,0.));
#33563=CARTESIAN_POINT('',(22.,-0.75,0.));
#33564=CARTESIAN_POINT('',(0.,-0.75,0.));
#33565=CARTESIAN_POINT('Origin',(0.,-0.75,0.85));
#33566=CARTESIAN_POINT('',(0.,-0.75,0.85));
#33567=CARTESIAN_POINT('',(22.,-0.75,0.85));
#33568=CARTESIAN_POINT('Origin',(22.,0.,0.75));
#33569=CARTESIAN_POINT('Origin',(0.,0.,0.75));
#62800=UNCERTAINTY_MEASURE_WITH_UNIT(LENGTH_MEASURE(0.001),#62985,
'DISTANCE_ACCURACY_VALUE',
'Maximum model space distance between geometric entities at asserted c
onnectivities');
#62885=UNCERTAINTY_MEASURE_WITH_UNIT(LENGTH_MEASURE(0.001),#62985,
'DISTANCE_ACCURACY_VALUE',
'Maximum model space distance between geometric entities at asserted c
onnectivities');
#62899=(
GEOMETRIC_REPRESENTATION_CONTEXT(3)
GLOBAL_UNCERTAINTY_ASSIGNED_CONTEXT((#62800))
GLOBAL_UNIT_ASSIGNED_CONTEXT((#62985,#62987,#62988))
REPRESENTATION_CONTEXT('','3D')
);
#62984=(
GEOMETRIC_REPRESENTATION_CONTEXT(3)
GLOBAL_UNCERTAINTY_ASSIGNED_CONTEXT((#62885))
GLOBAL_UNIT_ASSIGNED_CONTEXT((#62985,#62987,#62988))
REPRESENTATION_CONTEXT('','3D')
);
#62985=(
LENGTH_UNIT()
NAMED_UNIT(*)
SI_UNIT(.CENTI.,.METRE.)
);
#62987=(
NAMED_UNIT(*)
PLANE_ANGLE_UNIT()
SI_UNIT($,.RADIAN.)
);
#62988=(
NAMED_UNIT(*)
SI_UNIT($,.STERADIAN.)
SOLID_ANGLE_UNIT()
);
#63002=SHAPE_DEFINITION_REPRESENTATION(#63100,#63362);
#63100=PRODUCT_DEFINITION_SHAPE('',$,#63461);
#63362=SHAPE_REPRESENTATION('',(#24242),#62899);
#63447=PRODUCT_DEFINITION_CONTEXT('part definition',#63743,'design');
#63461=PRODUCT_DEFINITION('Linear Guide Rail - 15 mm, 220 mm Long',
'Linear Guide Rail - 15 mm, 220 mm Long',#63559,#63447);
#63559=PRODUCT_DEFINITION_FORMATION('',$,#63758);
#63743=APPLICATION_CONTEXT(
'Core Data for Automotive Mechanical Design Process');
#63744=PRODUCT_CONTEXT('part definition',#63743,'mechanical');
#63758=PRODUCT('Linear Guide Rail - 15 mm, 220 mm Long',
'Linear Guide Rail - 15 mm, 220 mm Long',
'Linear Guide Rail - 15 mm, 220 mm Long',(#63744));
#63899=COLOUR_RGB('Sky Blue',0.24,0.69,0.87);
#63900=FILL_AREA_STYLE_COLOUR('',#63899);
#63901=FILL_AREA_STYLE('',(#63900));
#63902=SURFACE_STYLE_FILL_AREA(#63901);
#63903=SURFACE_SIDE_STYLE('',(#63902));
#63904=SURFACE_STYLE_USAGE(.BOTH.,#63903);
#63905=PRESENTATION_STYLE_ASSIGNMENT((#63904));
ENDSEC;
END-ISO-10303-21;
